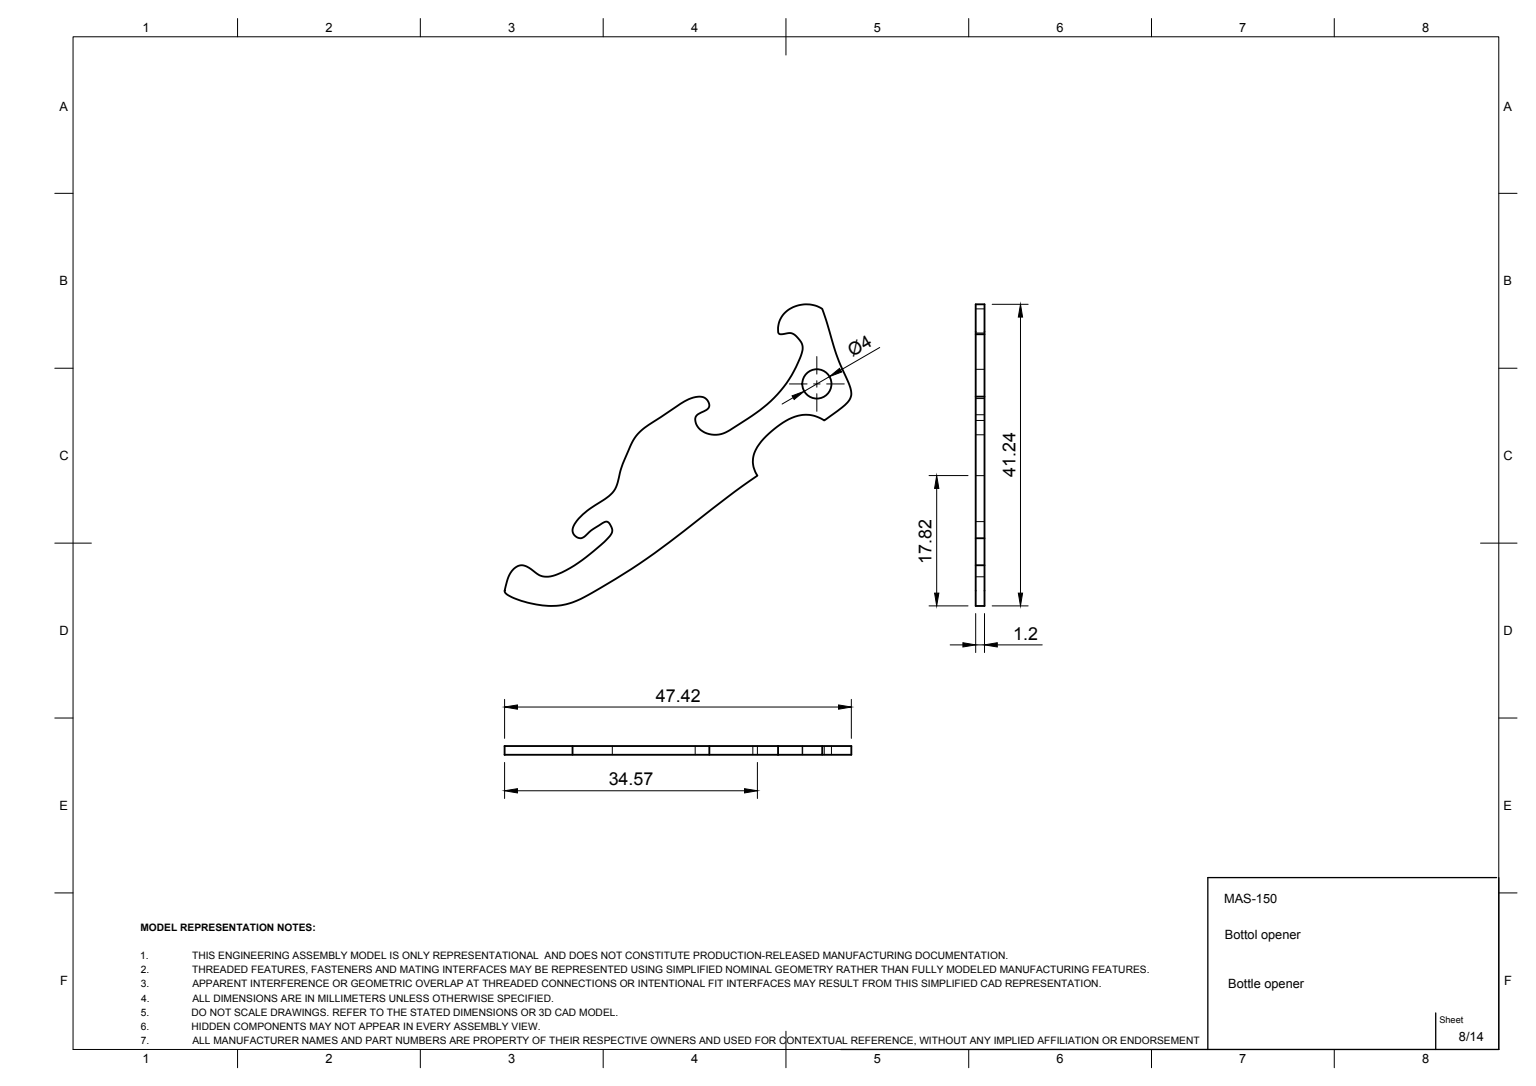
ISO-10303-21;
HEADER;
/* Generated by software containing ST-Developer
 * from STEP Tools, Inc. (www.steptools.com) 
 */

FILE_DESCRIPTION(
/* description */ ('STEP AP203'),
/* implementation_level */ '2;1');

FILE_NAME(
/* name */ 'Bottle opener.step',
/* time_stamp */ '2026-11-08T21:40:52-08:00',
/* author */ (''),
/* organization */ (''),
/* preprocessor_version */ 'ST-DEVELOPER v20.2',
/* originating_system */ 'Autodesk Translation Framework v15.17.0.0',
/* authorisation */ '');

FILE_SCHEMA (('AUTOMOTIVE_DESIGN { 1 0 10303 214 3 1 1 }'));
ENDSEC;

DATA;
#10=MECHANICAL_DESIGN_GEOMETRIC_PRESENTATION_REPRESENTATION('',(#190),#12137);
#128=B_SPLINE_CURVE_WITH_KNOTS('',3,(#11775,#11776,#11777,#11778,#11779,
#11780,#11781,#11782,#11783,#11784,#11785,#11786,#11787,#11788,#11789,#11790,
#11791,#11792,#11793,#11794,#11795,#11796,#11797,#11798,#11799,#11800,#11801,
#11802,#11803,#11804,#11805,#11806,#11807,#11808,#11809,#11810,#11811,#11812,
#11813,#11814,#11815,#11816,#11817,#11818),.UNSPECIFIED.,.F.,.F.,(4,1,1,
1,1,1,1,1,1,1,1,1,1,1,1,1,1,1,1,1,1,1,1,1,1,1,1,1,1,1,1,1,1,1,1,1,1,1,1,
1,1,4),(0.,0.0155086969164078,0.0371731810819821,0.0514015376726156,0.0721494932844473,
0.0879462852339701,0.102136934793609,0.118096046183078,0.19862023937012,
0.220465782155634,0.23365418085247,0.241548051822006,0.250379403180355,
0.265039089454663,0.283941482221575,0.302847655089067,0.314345531734621,
0.357463421988275,0.386547700128901,0.416631362178992,0.447827251721429,
0.480835486339271,0.507932786796811,0.529341861229807,0.553738573125003,
0.594012510221834,0.628912316880978,0.64568724667197,0.66015205447044,0.674349782601168,
0.687580075802142,0.700468884473892,0.724215901035998,0.747660515873313,
0.770169322257755,0.837047273198873,0.898018999477543,0.927421383188233,
0.952466294986228,0.96568815856341,0.980894474823001,1.),.UNSPECIFIED.);
#129=B_SPLINE_CURVE_WITH_KNOTS('',3,(#11822,#11823,#11824,#11825,#11826,
#11827,#11828,#11829,#11830,#11831,#11832,#11833,#11834,#11835,#11836,#11837,
#11838,#11839,#11840,#11841,#11842,#11843,#11844,#11845,#11846,#11847,#11848,
#11849,#11850,#11851,#11852,#11853,#11854,#11855,#11856,#11857,#11858,#11859,
#11860,#11861,#11862,#11863,#11864,#11865),.UNSPECIFIED.,.F.,.F.,(4,1,1,
1,1,1,1,1,1,1,1,1,1,1,1,1,1,1,1,1,1,1,1,1,1,1,1,1,1,1,1,1,1,1,1,1,1,1,1,
1,1,4),(0.,0.0155086969164078,0.0371731810819821,0.0514015376726156,0.0721494932844473,
0.0879462852339701,0.102136934793609,0.118096046183078,0.19862023937012,
0.220465782155634,0.23365418085247,0.241548051822006,0.250379403180355,
0.265039089454663,0.283941482221575,0.302847655089067,0.314345531734621,
0.357463421988275,0.386547700128901,0.416631362178992,0.447827251721429,
0.480835486339271,0.507932786796811,0.529341861229807,0.553738573125003,
0.594012510221834,0.628912316880978,0.64568724667197,0.66015205447044,0.674349782601168,
0.687580075802142,0.700468884473892,0.724215901035998,0.747660515873313,
0.770169322257755,0.837047273198873,0.898018999477543,0.927421383188233,
0.952466294986228,0.96568815856341,0.980894474823001,1.),.UNSPECIFIED.);
#130=B_SPLINE_CURVE_WITH_KNOTS('',3,(#11878,#11879,#11880,#11881),
 .UNSPECIFIED.,.F.,.F.,(4,4),(0.,1.),.UNSPECIFIED.);
#131=B_SPLINE_CURVE_WITH_KNOTS('',3,(#11884,#11885,#11886,#11887),
 .UNSPECIFIED.,.F.,.F.,(4,4),(0.,1.),.UNSPECIFIED.);
#132=B_SPLINE_CURVE_WITH_KNOTS('',3,(#11901,#11902,#11903,#11904,#11905,
#11906),.UNSPECIFIED.,.F.,.F.,(4,1,1,4),(0.,0.470503009353909,0.684670022609357,
1.),.UNSPECIFIED.);
#133=B_SPLINE_CURVE_WITH_KNOTS('',3,(#11909,#11910,#11911,#11912,#11913,
#11914),.UNSPECIFIED.,.F.,.F.,(4,1,1,4),(0.,0.470503009353909,0.684670022609357,
1.),.UNSPECIFIED.);
#134=B_SPLINE_CURVE_WITH_KNOTS('',3,(#11926,#11927,#11928,#11929,#11930),
 .UNSPECIFIED.,.F.,.F.,(4,1,4),(0.,0.519782906107891,1.),.UNSPECIFIED.);
#135=B_SPLINE_CURVE_WITH_KNOTS('',3,(#11933,#11934,#11935,#11936,#11937),
 .UNSPECIFIED.,.F.,.F.,(4,1,4),(0.,0.519782906107891,1.),.UNSPECIFIED.);
#136=B_SPLINE_CURVE_WITH_KNOTS('',3,(#11952,#11953,#11954,#11955,#11956,
#11957,#11958),.UNSPECIFIED.,.F.,.F.,(4,1,1,1,4),(0.,0.490961406160804,
0.688676820334042,0.846051539210629,1.),.UNSPECIFIED.);
#137=B_SPLINE_CURVE_WITH_KNOTS('',3,(#11959,#11960,#11961,#11962,#11963,
#11964,#11965),.UNSPECIFIED.,.F.,.F.,(4,1,1,1,4),(0.,0.490961406160804,
0.688676820334042,0.846051539210629,1.),.UNSPECIFIED.);
#156=B_SPLINE_SURFACE_WITH_KNOTS('',3,1,((#11685,#11686),(#11687,#11688),
(#11689,#11690),(#11691,#11692),(#11693,#11694),(#11695,#11696),(#11697,
#11698),(#11699,#11700),(#11701,#11702),(#11703,#11704),(#11705,#11706),
(#11707,#11708),(#11709,#11710),(#11711,#11712),(#11713,#11714),(#11715,
#11716),(#11717,#11718),(#11719,#11720),(#11721,#11722),(#11723,#11724),
(#11725,#11726),(#11727,#11728),(#11729,#11730),(#11731,#11732),(#11733,
#11734),(#11735,#11736),(#11737,#11738),(#11739,#11740),(#11741,#11742),
(#11743,#11744),(#11745,#11746),(#11747,#11748),(#11749,#11750),(#11751,
#11752),(#11753,#11754),(#11755,#11756),(#11757,#11758),(#11759,#11760),
(#11761,#11762),(#11763,#11764),(#11765,#11766),(#11767,#11768),(#11769,
#11770),(#11771,#11772)),.UNSPECIFIED.,.F.,.F.,.F.,(4,1,1,1,1,1,1,1,1,1,
1,1,1,1,1,1,1,1,1,1,1,1,1,1,1,1,1,1,1,1,1,1,1,1,1,1,1,1,1,1,1,4),(2,2),
(0.,0.0155086969164078,0.0371731810819821,0.0514015376726156,0.0721494932844473,
0.0879462852339701,0.102136934793609,0.118096046183078,0.19862023937012,
0.220465782155634,0.23365418085247,0.241548051822006,0.250379403180355,
0.265039089454663,0.283941482221575,0.302847655089067,0.314345531734621,
0.357463421988275,0.386547700128901,0.416631362178992,0.447827251721429,
0.480835486339271,0.507932786796811,0.529341861229807,0.553738573125003,
0.594012510221834,0.628912316880978,0.64568724667197,0.66015205447044,0.674349782601168,
0.687580075802142,0.700468884473892,0.724215901035998,0.747660515873313,
0.770169322257755,0.837047273198873,0.898018999477543,0.927421383188233,
0.952466294986228,0.96568815856341,0.980894474823001,1.),(0.,0.1728),
 .UNSPECIFIED.);
#157=B_SPLINE_SURFACE_WITH_KNOTS('',3,1,((#11867,#11868),(#11869,#11870),
(#11871,#11872),(#11873,#11874),(#11875,#11876)),.UNSPECIFIED.,.F.,.F.,
 .F.,(4,1,4),(2,2),(0.,0.376046516805316,1.),(0.,0.1728),.UNSPECIFIED.);
#158=B_SPLINE_SURFACE_WITH_KNOTS('',3,1,((#11888,#11889),(#11890,#11891),
(#11892,#11893),(#11894,#11895),(#11896,#11897),(#11898,#11899)),
 .UNSPECIFIED.,.F.,.F.,.F.,(4,1,1,4),(2,2),(0.,0.470503009353909,0.684670022609357,
1.),(0.,0.1728),.UNSPECIFIED.);
#159=B_SPLINE_SURFACE_WITH_KNOTS('',3,1,((#11915,#11916),(#11917,#11918),
(#11919,#11920),(#11921,#11922),(#11923,#11924)),.UNSPECIFIED.,.F.,.F.,
 .F.,(4,1,4),(2,2),(0.,0.519782906107891,1.),(0.,0.1728),.UNSPECIFIED.);
#160=B_SPLINE_SURFACE_WITH_KNOTS('',3,1,((#11938,#11939),(#11940,#11941),
(#11942,#11943),(#11944,#11945),(#11946,#11947),(#11948,#11949),(#11950,
#11951)),.UNSPECIFIED.,.F.,.F.,.F.,(4,1,1,1,4),(2,2),(0.,0.490961406160804,
0.688676820334042,0.846051539210629,1.),(0.,0.1728),.UNSPECIFIED.);
#168=SHAPE_REPRESENTATION_RELATIONSHIP('SRR','None',#12192,#179);
#179=ADVANCED_BREP_SHAPE_REPRESENTATION('',(#201),#12133);
#190=STYLED_ITEM('',(#12253),#201);
#201=MANIFOLD_SOLID_BREP('Body1',#1835);
#221=FACE_BOUND('',#696,.T.);
#222=FACE_BOUND('',#698,.T.);
#263=PLANE('',#2078);
#264=PLANE('',#2079);
#340=LINE('',#11683,#434);
#341=LINE('',#11820,#435);
#342=LINE('',#11866,#436);
#343=LINE('',#11883,#437);
#344=LINE('',#11908,#438);
#345=LINE('',#11932,#439);
#434=VECTOR('',#2456,2.00000000000001);
#435=VECTOR('',#2459,1000.);
#436=VECTOR('',#2460,1000.);
#437=VECTOR('',#2461,1000.);
#438=VECTOR('',#2462,1000.);
#439=VECTOR('',#2463,1000.);
#477=CYLINDRICAL_SURFACE('',#2075,2.00000000000001);
#563=FACE_OUTER_BOUND('',#689,.T.);
#564=FACE_OUTER_BOUND('',#690,.T.);
#565=FACE_OUTER_BOUND('',#691,.T.);
#566=FACE_OUTER_BOUND('',#692,.T.);
#567=FACE_OUTER_BOUND('',#693,.T.);
#568=FACE_OUTER_BOUND('',#694,.T.);
#569=FACE_OUTER_BOUND('',#695,.T.);
#570=FACE_OUTER_BOUND('',#697,.T.);
#689=EDGE_LOOP('',(#1551,#1552,#1553,#1554));
#690=EDGE_LOOP('',(#1555,#1556,#1557,#1558));
#691=EDGE_LOOP('',(#1559,#1560,#1561,#1562));
#692=EDGE_LOOP('',(#1563,#1564,#1565,#1566));
#693=EDGE_LOOP('',(#1567,#1568,#1569,#1570));
#694=EDGE_LOOP('',(#1571,#1572,#1573,#1574));
#695=EDGE_LOOP('',(#1575,#1576,#1577,#1578,#1579));
#696=EDGE_LOOP('',(#1580));
#697=EDGE_LOOP('',(#1581,#1582,#1583,#1584,#1585));
#698=EDGE_LOOP('',(#1586));
#786=CIRCLE('',#2076,2.00000000000001);
#787=CIRCLE('',#2077,2.00000000000001);
#931=VERTEX_POINT('',#11680);
#932=VERTEX_POINT('',#11682);
#933=VERTEX_POINT('',#11773);
#934=VERTEX_POINT('',#11774);
#935=VERTEX_POINT('',#11819);
#936=VERTEX_POINT('',#11821);
#937=VERTEX_POINT('',#11877);
#938=VERTEX_POINT('',#11882);
#939=VERTEX_POINT('',#11900);
#940=VERTEX_POINT('',#11907);
#941=VERTEX_POINT('',#11925);
#942=VERTEX_POINT('',#11931);
#1145=EDGE_CURVE('',#931,#931,#786,.T.);
#1146=EDGE_CURVE('',#931,#932,#340,.T.);
#1147=EDGE_CURVE('',#932,#932,#787,.T.);
#1148=EDGE_CURVE('',#933,#934,#128,.T.);
#1149=EDGE_CURVE('',#935,#934,#341,.T.);
#1150=EDGE_CURVE('',#936,#935,#129,.T.);
#1151=EDGE_CURVE('',#936,#933,#342,.T.);
#1152=EDGE_CURVE('',#934,#937,#130,.T.);
#1153=EDGE_CURVE('',#938,#937,#343,.T.);
#1154=EDGE_CURVE('',#935,#938,#131,.T.);
#1155=EDGE_CURVE('',#937,#939,#132,.T.);
#1156=EDGE_CURVE('',#940,#939,#344,.T.);
#1157=EDGE_CURVE('',#938,#940,#133,.T.);
#1158=EDGE_CURVE('',#939,#941,#134,.T.);
#1159=EDGE_CURVE('',#942,#941,#345,.T.);
#1160=EDGE_CURVE('',#940,#942,#135,.T.);
#1161=EDGE_CURVE('',#941,#933,#136,.T.);
#1162=EDGE_CURVE('',#942,#936,#137,.T.);
#1551=ORIENTED_EDGE('',*,*,#1145,.F.);
#1552=ORIENTED_EDGE('',*,*,#1146,.T.);
#1553=ORIENTED_EDGE('',*,*,#1147,.T.);
#1554=ORIENTED_EDGE('',*,*,#1146,.F.);
#1555=ORIENTED_EDGE('',*,*,#1148,.T.);
#1556=ORIENTED_EDGE('',*,*,#1149,.F.);
#1557=ORIENTED_EDGE('',*,*,#1150,.F.);
#1558=ORIENTED_EDGE('',*,*,#1151,.T.);
#1559=ORIENTED_EDGE('',*,*,#1152,.T.);
#1560=ORIENTED_EDGE('',*,*,#1153,.F.);
#1561=ORIENTED_EDGE('',*,*,#1154,.F.);
#1562=ORIENTED_EDGE('',*,*,#1149,.T.);
#1563=ORIENTED_EDGE('',*,*,#1155,.T.);
#1564=ORIENTED_EDGE('',*,*,#1156,.F.);
#1565=ORIENTED_EDGE('',*,*,#1157,.F.);
#1566=ORIENTED_EDGE('',*,*,#1153,.T.);
#1567=ORIENTED_EDGE('',*,*,#1158,.T.);
#1568=ORIENTED_EDGE('',*,*,#1159,.F.);
#1569=ORIENTED_EDGE('',*,*,#1160,.F.);
#1570=ORIENTED_EDGE('',*,*,#1156,.T.);
#1571=ORIENTED_EDGE('',*,*,#1161,.T.);
#1572=ORIENTED_EDGE('',*,*,#1151,.F.);
#1573=ORIENTED_EDGE('',*,*,#1162,.F.);
#1574=ORIENTED_EDGE('',*,*,#1159,.T.);
#1575=ORIENTED_EDGE('',*,*,#1150,.T.);
#1576=ORIENTED_EDGE('',*,*,#1154,.T.);
#1577=ORIENTED_EDGE('',*,*,#1157,.T.);
#1578=ORIENTED_EDGE('',*,*,#1160,.T.);
#1579=ORIENTED_EDGE('',*,*,#1162,.T.);
#1580=ORIENTED_EDGE('',*,*,#1147,.F.);
#1581=ORIENTED_EDGE('',*,*,#1148,.F.);
#1582=ORIENTED_EDGE('',*,*,#1161,.F.);
#1583=ORIENTED_EDGE('',*,*,#1158,.F.);
#1584=ORIENTED_EDGE('',*,*,#1155,.F.);
#1585=ORIENTED_EDGE('',*,*,#1152,.F.);
#1586=ORIENTED_EDGE('',*,*,#1145,.T.);
#1791=ADVANCED_FACE('',(#563),#477,.F.);
#1792=ADVANCED_FACE('',(#564),#156,.F.);
#1793=ADVANCED_FACE('',(#565),#157,.F.);
#1794=ADVANCED_FACE('',(#566),#158,.F.);
#1795=ADVANCED_FACE('',(#567),#159,.F.);
#1796=ADVANCED_FACE('',(#568),#160,.F.);
#1797=ADVANCED_FACE('',(#569,#221),#263,.T.);
#1798=ADVANCED_FACE('',(#570,#222),#264,.F.);
#1835=CLOSED_SHELL('',(#1791,#1792,#1793,#1794,#1795,#1796,#1797,#1798));
#2074=AXIS2_PLACEMENT_3D('',#11678,#2450,#2451);
#2075=AXIS2_PLACEMENT_3D('',#11679,#2452,#2453);
#2076=AXIS2_PLACEMENT_3D('',#11681,#2454,#2455);
#2077=AXIS2_PLACEMENT_3D('',#11684,#2457,#2458);
#2078=AXIS2_PLACEMENT_3D('',#11966,#2464,#2465);
#2079=AXIS2_PLACEMENT_3D('',#11967,#2466,#2467);
#2450=DIRECTION('axis',(0.,0.,1.));
#2451=DIRECTION('refdir',(1.,0.,0.));
#2452=DIRECTION('center_axis',(-1.77763333866942E-31,1.,8.62816615085482E-32));
#2453=DIRECTION('ref_axis',(2.87582171275097E-62,-8.62816615085482E-32,
1.));
#2454=DIRECTION('center_axis',(-1.77763333866942E-31,1.,8.62816615085482E-32));
#2455=DIRECTION('ref_axis',(2.87582171275097E-62,-8.62816615085482E-32,
1.));
#2456=DIRECTION('',(-1.77763333866942E-31,1.,8.62816615085482E-32));
#2457=DIRECTION('center_axis',(-1.77763333866942E-31,1.,8.62816615085482E-32));
#2458=DIRECTION('ref_axis',(1.53377158013385E-62,-8.62816615085482E-32,
1.));
#2459=DIRECTION('',(1.77763333866942E-31,-1.,-8.62816615085482E-32));
#2460=DIRECTION('',(1.77763333866942E-31,-1.,-8.62816615085482E-32));
#2461=DIRECTION('',(1.77763333866942E-31,-1.,-8.62816615085482E-32));
#2462=DIRECTION('',(1.77763333866942E-31,-1.,-8.62816615085482E-32));
#2463=DIRECTION('',(1.77763333866942E-31,-1.,-8.62816615085482E-32));
#2464=DIRECTION('center_axis',(-1.77763333866942E-31,1.,-7.54964538199795E-32));
#2465=DIRECTION('ref_axis',(2.67771827758074E-79,7.54964538199795E-32,1.));
#2466=DIRECTION('center_axis',(-1.77763333866942E-31,1.,-7.54964538199795E-32));
#2467=DIRECTION('ref_axis',(2.67771827758074E-79,7.54964538199795E-32,1.));
#11678=CARTESIAN_POINT('',(0.,0.,0.));
#11679=CARTESIAN_POINT('Origin',(22.9603057217174,0.,-2.33853588412019));
#11680=CARTESIAN_POINT('',(22.9603057217174,1.72563323017097E-31,-4.3385358841202));
#11681=CARTESIAN_POINT('Origin',(22.9603057217174,0.,-2.33853588412019));
#11682=CARTESIAN_POINT('',(22.9603057217174,1.2,-4.3385358841202));
#11683=CARTESIAN_POINT('',(22.9603057217174,1.72563323017097E-31,-4.3385358841202));
#11684=CARTESIAN_POINT('Origin',(22.9603057217174,1.2,-2.33853588412019));
#11685=CARTESIAN_POINT('Ctrl Pts',(-28.2500418808544,1.2,-2.07888836971772));
#11686=CARTESIAN_POINT('Ctrl Pts',(-28.2500418808544,-0.527999999999998,
-2.07888836971772));
#11687=CARTESIAN_POINT('Ctrl Pts',(-27.9613439331009,1.2,-1.81555449964671));
#11688=CARTESIAN_POINT('Ctrl Pts',(-27.9613439331009,-0.527999999999998,
-1.81555449964671));
#11689=CARTESIAN_POINT('Ctrl Pts',(-27.180603234679,1.2,-1.04385836116026));
#11690=CARTESIAN_POINT('Ctrl Pts',(-27.180603234679,-0.527999999999998,
-1.04385836116026));
#11691=CARTESIAN_POINT('Ctrl Pts',(-25.9983030006616,1.2,-0.24124876693352));
#11692=CARTESIAN_POINT('Ctrl Pts',(-25.9983030006616,-0.527999999999998,
-0.24124876693352));
#11693=CARTESIAN_POINT('Ctrl Pts',(-24.2346861695509,1.2,-0.210983790359477));
#11694=CARTESIAN_POINT('Ctrl Pts',(-24.2346861695509,-0.527999999999998,
-0.210983790359477));
#11695=CARTESIAN_POINT('Ctrl Pts',(-23.517870169039,1.2,-1.68305705631707));
#11696=CARTESIAN_POINT('Ctrl Pts',(-23.517870169039,-0.527999999999998,
-1.68305705631707));
#11697=CARTESIAN_POINT('Ctrl Pts',(-23.2233109717715,1.2,-3.05602157557454));
#11698=CARTESIAN_POINT('Ctrl Pts',(-23.2233109717715,-0.527999999999998,
-3.05602157557454));
#11699=CARTESIAN_POINT('Ctrl Pts',(-22.1784263046757,1.2,-3.93337248074442));
#11700=CARTESIAN_POINT('Ctrl Pts',(-22.1784263046757,-0.527999999999998,
-3.93337248074442));
#11701=CARTESIAN_POINT('Ctrl Pts',(-19.19441431546,1.2,-4.74815122044273));
#11702=CARTESIAN_POINT('Ctrl Pts',(-19.19441431546,-0.527999999999998,-4.74815122044273));
#11703=CARTESIAN_POINT('Ctrl Pts',(-15.7509580358841,1.2,-4.44216895895114));
#11704=CARTESIAN_POINT('Ctrl Pts',(-15.7509580358841,-0.527999999999998,
-4.44216895895114));
#11705=CARTESIAN_POINT('Ctrl Pts',(-12.7021174144063,1.2,-4.06331666259747));
#11706=CARTESIAN_POINT('Ctrl Pts',(-12.7021174144063,-0.527999999999998,
-4.06331666259747));
#11707=CARTESIAN_POINT('Ctrl Pts',(-11.3962777017639,1.2,-3.64648316501468));
#11708=CARTESIAN_POINT('Ctrl Pts',(-11.3962777017639,-0.527999999999998,
-3.64648316501468));
#11709=CARTESIAN_POINT('Ctrl Pts',(-11.2344759364774,1.2,-2.80455171594097));
#11710=CARTESIAN_POINT('Ctrl Pts',(-11.2344759364774,-0.527999999999998,
-2.80455171594097));
#11711=CARTESIAN_POINT('Ctrl Pts',(-11.1732737269437,1.2,-1.7662619507528));
#11712=CARTESIAN_POINT('Ctrl Pts',(-11.1732737269437,-0.527999999999998,
-1.7662619507528));
#11713=CARTESIAN_POINT('Ctrl Pts',(-12.7612302838612,1.2,-1.89361059761595));
#11714=CARTESIAN_POINT('Ctrl Pts',(-12.7612302838612,-0.527999999999998,
-1.89361059761595));
#11715=CARTESIAN_POINT('Ctrl Pts',(-13.9972305202523,1.2,-1.67844839769156));
#11716=CARTESIAN_POINT('Ctrl Pts',(-13.9972305202523,-0.527999999999998,
-1.67844839769156));
#11717=CARTESIAN_POINT('Ctrl Pts',(-15.6400181726054,1.2,-2.29491586659866));
#11718=CARTESIAN_POINT('Ctrl Pts',(-15.6400181726054,-0.527999999999998,
-2.29491586659866));
#11719=CARTESIAN_POINT('Ctrl Pts',(-16.7051564115516,1.2,0.0418535888021335));
#11720=CARTESIAN_POINT('Ctrl Pts',(-16.7051564115516,-0.527999999999998,
0.0418535888021335));
#11721=CARTESIAN_POINT('Ctrl Pts',(-13.0664970088623,1.2,0.88071809162054));
#11722=CARTESIAN_POINT('Ctrl Pts',(-13.0664970088623,-0.527999999999998,
0.88071809162054));
#11723=CARTESIAN_POINT('Ctrl Pts',(-10.5984973129989,1.2,0.680667707785562));
#11724=CARTESIAN_POINT('Ctrl Pts',(-10.5984973129989,-0.527999999999998,
0.680667707785562));
#11725=CARTESIAN_POINT('Ctrl Pts',(-7.82942308877726,1.2,0.695565326486597));
#11726=CARTESIAN_POINT('Ctrl Pts',(-7.82942308877726,-0.527999999999998,
0.695565326486597));
#11727=CARTESIAN_POINT('Ctrl Pts',(-6.07620266579566,1.2,2.85997113365485));
#11728=CARTESIAN_POINT('Ctrl Pts',(-6.07620266579566,-0.527999999999998,
2.85997113365485));
#11729=CARTESIAN_POINT('Ctrl Pts',(-3.9066933893458,1.2,4.14091208560258));
#11730=CARTESIAN_POINT('Ctrl Pts',(-3.9066933893458,-0.527999999999998,
4.14091208560258));
#11731=CARTESIAN_POINT('Ctrl Pts',(-2.0279101215411,1.2,5.46819912841997));
#11732=CARTESIAN_POINT('Ctrl Pts',(-2.0279101215411,-0.527999999999998,
5.46819912841997));
#11733=CARTESIAN_POINT('Ctrl Pts',(0.00386116068497311,1.2,5.86471136207473));
#11734=CARTESIAN_POINT('Ctrl Pts',(0.00386116068497311,-0.527999999999998,
5.86471136207473));
#11735=CARTESIAN_POINT('Ctrl Pts',(2.39576994688095,1.2,5.73794061249253));
#11736=CARTESIAN_POINT('Ctrl Pts',(2.39576994688095,-0.527999999999998,
5.73794061249253));
#11737=CARTESIAN_POINT('Ctrl Pts',(5.15590481840992,1.2,5.78580883625202));
#11738=CARTESIAN_POINT('Ctrl Pts',(5.15590481840992,-0.527999999999998,
5.78580883625202));
#11739=CARTESIAN_POINT('Ctrl Pts',(7.73518803149787,1.2,5.79127386586831));
#11740=CARTESIAN_POINT('Ctrl Pts',(7.73518803149787,-0.527999999999998,
5.79127386586831));
#11741=CARTESIAN_POINT('Ctrl Pts',(9.45734572072178,1.2,4.67363967594622));
#11742=CARTESIAN_POINT('Ctrl Pts',(9.45734572072178,-0.527999999999998,
4.67363967594622));
#11743=CARTESIAN_POINT('Ctrl Pts',(9.17706365495184,1.2,2.96306509995752));
#11744=CARTESIAN_POINT('Ctrl Pts',(9.17706365495184,-0.527999999999998,
2.96306509995752));
#11745=CARTESIAN_POINT('Ctrl Pts',(7.81796360098053,1.2,3.18513163158631));
#11746=CARTESIAN_POINT('Ctrl Pts',(7.81796360098053,-0.527999999999998,
3.18513163158631));
#11747=CARTESIAN_POINT('Ctrl Pts',(6.59699346312693,1.2,3.38520430984983));
#11748=CARTESIAN_POINT('Ctrl Pts',(6.59699346312693,-0.527999999999998,
3.38520430984983));
#11749=CARTESIAN_POINT('Ctrl Pts',(5.93021602745299,1.2,1.85802575211607));
#11750=CARTESIAN_POINT('Ctrl Pts',(5.93021602745299,-0.527999999999998,
1.85802575211607));
#11751=CARTESIAN_POINT('Ctrl Pts',(6.62071623580517,1.2,0.188782666588939));
#11752=CARTESIAN_POINT('Ctrl Pts',(6.62071623580517,-0.527999999999998,
0.188782666588939));
#11753=CARTESIAN_POINT('Ctrl Pts',(8.32325294445203,1.2,-0.970953886492654));
#11754=CARTESIAN_POINT('Ctrl Pts',(8.32325294445203,-0.527999999999998,
-0.970953886492654));
#11755=CARTESIAN_POINT('Ctrl Pts',(11.5219206080117,1.2,-0.983963678117389));
#11756=CARTESIAN_POINT('Ctrl Pts',(11.5219206080117,-0.527999999999998,
-0.983963678117389));
#11757=CARTESIAN_POINT('Ctrl Pts',(15.6615569014707,1.2,-1.18440486857005));
#11758=CARTESIAN_POINT('Ctrl Pts',(15.6615569014707,-0.527999999999998,
-1.18440486857005));
#11759=CARTESIAN_POINT('Ctrl Pts',(20.0374444881341,1.2,0.065252622484184));
#11760=CARTESIAN_POINT('Ctrl Pts',(20.0374444881341,-0.527999999999998,
0.065252622484184));
#11761=CARTESIAN_POINT('Ctrl Pts',(22.6903241895972,1.2,1.63809077991409));
#11762=CARTESIAN_POINT('Ctrl Pts',(22.6903241895972,-0.527999999999998,
1.63809077991409));
#11763=CARTESIAN_POINT('Ctrl Pts',(24.4689719714588,1.2,2.87083584760694));
#11764=CARTESIAN_POINT('Ctrl Pts',(24.4689719714588,-0.527999999999998,
2.87083584760694));
#11765=CARTESIAN_POINT('Ctrl Pts',(24.3083816239237,1.2,4.43315301466272));
#11766=CARTESIAN_POINT('Ctrl Pts',(24.3083816239237,-0.527999999999998,
4.43315301466272));
#11767=CARTESIAN_POINT('Ctrl Pts',(24.0522028467612,1.2,5.77390669222975));
#11768=CARTESIAN_POINT('Ctrl Pts',(24.0522028467612,-0.527999999999998,
5.77390669222975));
#11769=CARTESIAN_POINT('Ctrl Pts',(22.2137376328105,1.2,5.96195834426836));
#11770=CARTESIAN_POINT('Ctrl Pts',(22.2137376328105,-0.527999999999998,
5.96195834426836));
#11771=CARTESIAN_POINT('Ctrl Pts',(22.5278884970739,1.2,6.53446701068235));
#11772=CARTESIAN_POINT('Ctrl Pts',(22.5278884970739,-0.527999999999998,
6.53446701068235));
#11773=CARTESIAN_POINT('',(-28.2500418808543,0.,-2.07888836971769));
#11774=CARTESIAN_POINT('',(22.5278884970739,0.,6.53446701068235));
#11775=CARTESIAN_POINT('Ctrl Pts',(-28.2500418808543,0.,-2.07888836971769));
#11776=CARTESIAN_POINT('Ctrl Pts',(-27.9613439331009,0.,-1.81555449964671));
#11777=CARTESIAN_POINT('Ctrl Pts',(-27.180603234679,0.,-1.04385836116026));
#11778=CARTESIAN_POINT('Ctrl Pts',(-25.9983030006616,0.,-0.24124876693352));
#11779=CARTESIAN_POINT('Ctrl Pts',(-24.2346861695509,0.,-0.210983790359477));
#11780=CARTESIAN_POINT('Ctrl Pts',(-23.517870169039,0.,-1.68305705631707));
#11781=CARTESIAN_POINT('Ctrl Pts',(-23.2233109717715,0.,-3.05602157557454));
#11782=CARTESIAN_POINT('Ctrl Pts',(-22.1784263046757,0.,-3.93337248074442));
#11783=CARTESIAN_POINT('Ctrl Pts',(-19.19441431546,0.,-4.74815122044273));
#11784=CARTESIAN_POINT('Ctrl Pts',(-15.7509580358841,0.,-4.44216895895114));
#11785=CARTESIAN_POINT('Ctrl Pts',(-12.7021174144063,0.,-4.06331666259747));
#11786=CARTESIAN_POINT('Ctrl Pts',(-11.3962777017639,0.,-3.64648316501468));
#11787=CARTESIAN_POINT('Ctrl Pts',(-11.2344759364774,0.,-2.80455171594097));
#11788=CARTESIAN_POINT('Ctrl Pts',(-11.1732737269437,0.,-1.7662619507528));
#11789=CARTESIAN_POINT('Ctrl Pts',(-12.7612302838612,0.,-1.89361059761595));
#11790=CARTESIAN_POINT('Ctrl Pts',(-13.9972305202523,0.,-1.67844839769156));
#11791=CARTESIAN_POINT('Ctrl Pts',(-15.6400181726054,0.,-2.29491586659866));
#11792=CARTESIAN_POINT('Ctrl Pts',(-16.7051564115516,0.,0.0418535888021335));
#11793=CARTESIAN_POINT('Ctrl Pts',(-13.0664970088623,0.,0.88071809162054));
#11794=CARTESIAN_POINT('Ctrl Pts',(-10.5984973129989,0.,0.680667707785562));
#11795=CARTESIAN_POINT('Ctrl Pts',(-7.82942308877726,0.,0.695565326486597));
#11796=CARTESIAN_POINT('Ctrl Pts',(-6.07620266579566,0.,2.85997113365485));
#11797=CARTESIAN_POINT('Ctrl Pts',(-3.9066933893458,0.,4.14091208560258));
#11798=CARTESIAN_POINT('Ctrl Pts',(-2.0279101215411,0.,5.46819912841997));
#11799=CARTESIAN_POINT('Ctrl Pts',(0.00386116068497311,0.,5.86471136207473));
#11800=CARTESIAN_POINT('Ctrl Pts',(2.39576994688095,0.,5.73794061249253));
#11801=CARTESIAN_POINT('Ctrl Pts',(5.15590481840992,0.,5.78580883625202));
#11802=CARTESIAN_POINT('Ctrl Pts',(7.73518803149787,0.,5.79127386586831));
#11803=CARTESIAN_POINT('Ctrl Pts',(9.45734572072178,0.,4.67363967594622));
#11804=CARTESIAN_POINT('Ctrl Pts',(9.17706365495184,0.,2.96306509995752));
#11805=CARTESIAN_POINT('Ctrl Pts',(7.81796360098053,0.,3.18513163158631));
#11806=CARTESIAN_POINT('Ctrl Pts',(6.59699346312693,0.,3.38520430984983));
#11807=CARTESIAN_POINT('Ctrl Pts',(5.93021602745299,0.,1.85802575211607));
#11808=CARTESIAN_POINT('Ctrl Pts',(6.62071623580517,0.,0.188782666588939));
#11809=CARTESIAN_POINT('Ctrl Pts',(8.32325294445203,0.,-0.970953886492654));
#11810=CARTESIAN_POINT('Ctrl Pts',(11.5219206080117,0.,-0.983963678117389));
#11811=CARTESIAN_POINT('Ctrl Pts',(15.6615569014707,0.,-1.18440486857005));
#11812=CARTESIAN_POINT('Ctrl Pts',(20.0374444881341,0.,0.065252622484184));
#11813=CARTESIAN_POINT('Ctrl Pts',(22.6903241895972,0.,1.63809077991409));
#11814=CARTESIAN_POINT('Ctrl Pts',(24.4689719714588,0.,2.87083584760694));
#11815=CARTESIAN_POINT('Ctrl Pts',(24.3083816239237,0.,4.43315301466272));
#11816=CARTESIAN_POINT('Ctrl Pts',(24.0522028467612,0.,5.77390669222975));
#11817=CARTESIAN_POINT('Ctrl Pts',(22.2137376328105,0.,5.96195834426836));
#11818=CARTESIAN_POINT('Ctrl Pts',(22.5278884970739,0.,6.53446701068235));
#11819=CARTESIAN_POINT('',(22.5278884970739,1.2,6.53446701068235));
#11820=CARTESIAN_POINT('',(22.5278884970739,1.2,6.53446701068235));
#11821=CARTESIAN_POINT('',(-28.2500418808543,1.2,-2.07888836971769));
#11822=CARTESIAN_POINT('Ctrl Pts',(-28.2500418808543,1.2,-2.07888836971769));
#11823=CARTESIAN_POINT('Ctrl Pts',(-27.9613439331009,1.2,-1.81555449964671));
#11824=CARTESIAN_POINT('Ctrl Pts',(-27.180603234679,1.2,-1.04385836116026));
#11825=CARTESIAN_POINT('Ctrl Pts',(-25.9983030006616,1.2,-0.24124876693352));
#11826=CARTESIAN_POINT('Ctrl Pts',(-24.2346861695509,1.2,-0.210983790359477));
#11827=CARTESIAN_POINT('Ctrl Pts',(-23.517870169039,1.2,-1.68305705631707));
#11828=CARTESIAN_POINT('Ctrl Pts',(-23.2233109717715,1.2,-3.05602157557454));
#11829=CARTESIAN_POINT('Ctrl Pts',(-22.1784263046757,1.2,-3.93337248074442));
#11830=CARTESIAN_POINT('Ctrl Pts',(-19.19441431546,1.2,-4.74815122044273));
#11831=CARTESIAN_POINT('Ctrl Pts',(-15.7509580358841,1.2,-4.44216895895114));
#11832=CARTESIAN_POINT('Ctrl Pts',(-12.7021174144063,1.2,-4.06331666259747));
#11833=CARTESIAN_POINT('Ctrl Pts',(-11.3962777017639,1.2,-3.64648316501468));
#11834=CARTESIAN_POINT('Ctrl Pts',(-11.2344759364774,1.2,-2.80455171594097));
#11835=CARTESIAN_POINT('Ctrl Pts',(-11.1732737269437,1.2,-1.7662619507528));
#11836=CARTESIAN_POINT('Ctrl Pts',(-12.7612302838612,1.2,-1.89361059761595));
#11837=CARTESIAN_POINT('Ctrl Pts',(-13.9972305202523,1.2,-1.67844839769156));
#11838=CARTESIAN_POINT('Ctrl Pts',(-15.6400181726054,1.2,-2.29491586659866));
#11839=CARTESIAN_POINT('Ctrl Pts',(-16.7051564115516,1.2,0.0418535888021335));
#11840=CARTESIAN_POINT('Ctrl Pts',(-13.0664970088623,1.2,0.88071809162054));
#11841=CARTESIAN_POINT('Ctrl Pts',(-10.5984973129989,1.2,0.680667707785562));
#11842=CARTESIAN_POINT('Ctrl Pts',(-7.82942308877726,1.2,0.695565326486597));
#11843=CARTESIAN_POINT('Ctrl Pts',(-6.07620266579566,1.2,2.85997113365485));
#11844=CARTESIAN_POINT('Ctrl Pts',(-3.9066933893458,1.2,4.14091208560258));
#11845=CARTESIAN_POINT('Ctrl Pts',(-2.0279101215411,1.2,5.46819912841997));
#11846=CARTESIAN_POINT('Ctrl Pts',(0.00386116068497311,1.2,5.86471136207473));
#11847=CARTESIAN_POINT('Ctrl Pts',(2.39576994688095,1.2,5.73794061249253));
#11848=CARTESIAN_POINT('Ctrl Pts',(5.15590481840992,1.2,5.78580883625202));
#11849=CARTESIAN_POINT('Ctrl Pts',(7.73518803149787,1.2,5.79127386586831));
#11850=CARTESIAN_POINT('Ctrl Pts',(9.45734572072178,1.2,4.67363967594622));
#11851=CARTESIAN_POINT('Ctrl Pts',(9.17706365495184,1.2,2.96306509995752));
#11852=CARTESIAN_POINT('Ctrl Pts',(7.81796360098053,1.2,3.18513163158631));
#11853=CARTESIAN_POINT('Ctrl Pts',(6.59699346312693,1.2,3.38520430984983));
#11854=CARTESIAN_POINT('Ctrl Pts',(5.93021602745299,1.2,1.85802575211607));
#11855=CARTESIAN_POINT('Ctrl Pts',(6.62071623580517,1.2,0.188782666588939));
#11856=CARTESIAN_POINT('Ctrl Pts',(8.32325294445203,1.2,-0.970953886492654));
#11857=CARTESIAN_POINT('Ctrl Pts',(11.5219206080117,1.2,-0.983963678117389));
#11858=CARTESIAN_POINT('Ctrl Pts',(15.6615569014707,1.2,-1.18440486857005));
#11859=CARTESIAN_POINT('Ctrl Pts',(20.0374444881341,1.2,0.065252622484184));
#11860=CARTESIAN_POINT('Ctrl Pts',(22.6903241895972,1.2,1.63809077991409));
#11861=CARTESIAN_POINT('Ctrl Pts',(24.4689719714588,1.2,2.87083584760694));
#11862=CARTESIAN_POINT('Ctrl Pts',(24.3083816239237,1.2,4.43315301466272));
#11863=CARTESIAN_POINT('Ctrl Pts',(24.0522028467612,1.2,5.77390669222975));
#11864=CARTESIAN_POINT('Ctrl Pts',(22.2137376328105,1.2,5.96195834426836));
#11865=CARTESIAN_POINT('Ctrl Pts',(22.5278884970739,1.2,6.53446701068235));
#11866=CARTESIAN_POINT('',(-28.2500418808543,1.2,-2.07888836971769));
#11867=CARTESIAN_POINT('Ctrl Pts',(22.5278884970739,1.2,6.53446701068235));
#11868=CARTESIAN_POINT('Ctrl Pts',(22.5278884970739,-0.528,6.53446701068235));
#11869=CARTESIAN_POINT('Ctrl Pts',(23.1169295329987,1.2,7.60793564089319));
#11870=CARTESIAN_POINT('Ctrl Pts',(23.1169295329987,-0.528,7.60793564089319));
#11871=CARTESIAN_POINT('Ctrl Pts',(25.6536230216728,1.2,8.99671226634374));
#11872=CARTESIAN_POINT('Ctrl Pts',(25.6536230216728,-0.528,8.99671226634374));
#11873=CARTESIAN_POINT('Ctrl Pts',(28.6313409150419,1.2,7.38059742138985));
#11874=CARTESIAN_POINT('Ctrl Pts',(28.6313409150419,-0.528,7.38059742138985));
#11875=CARTESIAN_POINT('Ctrl Pts',(29.2791218831689,1.2,5.77930198399101));
#11876=CARTESIAN_POINT('Ctrl Pts',(29.2791218831689,-0.528,5.77930198399101));
#11877=CARTESIAN_POINT('',(29.2791218831689,0.,5.77930198399101));
#11878=CARTESIAN_POINT('Ctrl Pts',(22.5278884970739,0.,6.53446701068235));
#11879=CARTESIAN_POINT('Ctrl Pts',(24.0942932092593,0.,9.38908361325172));
#11880=CARTESIAN_POINT('Ctrl Pts',(28.2409339643995,0.,8.34567188259311));
#11881=CARTESIAN_POINT('Ctrl Pts',(29.2791218831689,0.,5.77930198399101));
#11882=CARTESIAN_POINT('',(29.2791218831689,1.2,5.77930198399101));
#11883=CARTESIAN_POINT('',(29.2791218831689,1.2,5.77930198399101));
#11884=CARTESIAN_POINT('Ctrl Pts',(22.5278884970739,1.2,6.53446701068235));
#11885=CARTESIAN_POINT('Ctrl Pts',(24.0942932092593,1.2,9.38908361325172));
#11886=CARTESIAN_POINT('Ctrl Pts',(28.2409339643995,1.2,8.34567188259311));
#11887=CARTESIAN_POINT('Ctrl Pts',(29.2791218831689,1.2,5.77930198399101));
#11888=CARTESIAN_POINT('Ctrl Pts',(29.2791218831689,1.2,5.77930198399101));
#11889=CARTESIAN_POINT('Ctrl Pts',(29.2791218831689,-0.528,5.77930198399101));
#11890=CARTESIAN_POINT('Ctrl Pts',(28.6578105275465,1.2,2.99017303105976));
#11891=CARTESIAN_POINT('Ctrl Pts',(28.6578105275465,-0.528,2.99017303105976));
#11892=CARTESIAN_POINT('Ctrl Pts',(27.094379352357,1.2,-0.177553803652863));
#11893=CARTESIAN_POINT('Ctrl Pts',(27.094379352357,-0.528,-0.177553803652863));
#11894=CARTESIAN_POINT('Ctrl Pts',(26.5382228845289,1.2,-7.0166851266602));
#11895=CARTESIAN_POINT('Ctrl Pts',(26.5382228845289,-0.528,-7.0166851266602));
#11896=CARTESIAN_POINT('Ctrl Pts',(24.629125296679,1.2,-6.94685713119016));
#11897=CARTESIAN_POINT('Ctrl Pts',(24.629125296679,-0.528,-6.94685713119016));
#11898=CARTESIAN_POINT('Ctrl Pts',(21.0225256793385,1.2,-7.04790997553116));
#11899=CARTESIAN_POINT('Ctrl Pts',(21.0225256793385,-0.528,-7.04790997553116));
#11900=CARTESIAN_POINT('',(21.0225256793385,0.,-7.04790997553116));
#11901=CARTESIAN_POINT('Ctrl Pts',(29.2791218831689,0.,5.77930198399101));
#11902=CARTESIAN_POINT('Ctrl Pts',(28.6578105275465,0.,2.99017303105976));
#11903=CARTESIAN_POINT('Ctrl Pts',(27.094379352357,0.,-0.177553803652863));
#11904=CARTESIAN_POINT('Ctrl Pts',(26.5382228845289,0.,-7.0166851266602));
#11905=CARTESIAN_POINT('Ctrl Pts',(24.629125296679,0.,-6.94685713119016));
#11906=CARTESIAN_POINT('Ctrl Pts',(21.0225256793385,0.,-7.04790997553116));
#11907=CARTESIAN_POINT('',(21.0225256793385,1.2,-7.04790997553116));
#11908=CARTESIAN_POINT('',(21.0225256793385,1.2,-7.04790997553116));
#11909=CARTESIAN_POINT('Ctrl Pts',(29.2791218831689,1.2,5.77930198399101));
#11910=CARTESIAN_POINT('Ctrl Pts',(28.6578105275465,1.2,2.99017303105976));
#11911=CARTESIAN_POINT('Ctrl Pts',(27.094379352357,1.2,-0.177553803652863));
#11912=CARTESIAN_POINT('Ctrl Pts',(26.5382228845289,1.2,-7.0166851266602));
#11913=CARTESIAN_POINT('Ctrl Pts',(24.629125296679,1.2,-6.94685713119016));
#11914=CARTESIAN_POINT('Ctrl Pts',(21.0225256793385,1.2,-7.04790997553116));
#11915=CARTESIAN_POINT('Ctrl Pts',(21.0225256793385,1.2,-7.04790997553116));
#11916=CARTESIAN_POINT('Ctrl Pts',(21.0225256793385,-0.528,-7.04790997553116));
#11917=CARTESIAN_POINT('Ctrl Pts',(19.8072013377325,1.2,-4.22629716477465));
#11918=CARTESIAN_POINT('Ctrl Pts',(19.8072013377325,-0.528,-4.22629716477465));
#11919=CARTESIAN_POINT('Ctrl Pts',(14.6387365156322,1.2,-3.68706222835893));
#11920=CARTESIAN_POINT('Ctrl Pts',(14.6387365156322,-0.528,-3.68706222835893));
#11921=CARTESIAN_POINT('Ctrl Pts',(9.29823038687031,1.2,-5.29769106666559));
#11922=CARTESIAN_POINT('Ctrl Pts',(9.29823038687031,-0.528,-5.29769106666559));
#11923=CARTESIAN_POINT('Ctrl Pts',(9.22738824529516,1.2,-8.22742371893551));
#11924=CARTESIAN_POINT('Ctrl Pts',(9.22738824529516,-0.528,-8.22742371893551));
#11925=CARTESIAN_POINT('',(9.22738824529516,0.,-8.22742371893551));
#11926=CARTESIAN_POINT('Ctrl Pts',(21.0225256793385,0.,-7.04790997553116));
#11927=CARTESIAN_POINT('Ctrl Pts',(19.8072013377325,0.,-4.22629716477465));
#11928=CARTESIAN_POINT('Ctrl Pts',(14.6387365156322,0.,-3.68706222835893));
#11929=CARTESIAN_POINT('Ctrl Pts',(9.29823038687031,0.,-5.29769106666559));
#11930=CARTESIAN_POINT('Ctrl Pts',(9.22738824529516,0.,-8.22742371893551));
#11931=CARTESIAN_POINT('',(9.22738824529516,1.2,-8.22742371893551));
#11932=CARTESIAN_POINT('',(9.22738824529516,1.2,-8.22742371893551));
#11933=CARTESIAN_POINT('Ctrl Pts',(21.0225256793385,1.2,-7.04790997553116));
#11934=CARTESIAN_POINT('Ctrl Pts',(19.8072013377325,1.2,-4.22629716477465));
#11935=CARTESIAN_POINT('Ctrl Pts',(14.6387365156322,1.2,-3.68706222835893));
#11936=CARTESIAN_POINT('Ctrl Pts',(9.29823038687031,1.2,-5.29769106666559));
#11937=CARTESIAN_POINT('Ctrl Pts',(9.22738824529516,1.2,-8.22742371893551));
#11938=CARTESIAN_POINT('Ctrl Pts',(9.22738824529516,1.2,-8.22742371893551));
#11939=CARTESIAN_POINT('Ctrl Pts',(9.22738824529516,-0.528,-8.22742371893551));
#11940=CARTESIAN_POINT('Ctrl Pts',(2.56764530386917,1.2,-8.25470956501187));
#11941=CARTESIAN_POINT('Ctrl Pts',(2.56764530386917,-0.528,-8.25470956501187));
#11942=CARTESIAN_POINT('Ctrl Pts',(-6.44753895416279,1.2,-9.5997804768992));
#11943=CARTESIAN_POINT('Ctrl Pts',(-6.44753895416279,-0.528,-9.5997804768992));
#11944=CARTESIAN_POINT('Ctrl Pts',(-18.1106375247657,1.2,-9.04522729065686));
#11945=CARTESIAN_POINT('Ctrl Pts',(-18.1106375247657,-0.528,-9.04522729065686));
#11946=CARTESIAN_POINT('Ctrl Pts',(-24.3161185416941,1.2,-8.46111575838443));
#11947=CARTESIAN_POINT('Ctrl Pts',(-24.3161185416941,-0.528,-8.46111575838443));
#11948=CARTESIAN_POINT('Ctrl Pts',(-28.8091126301565,1.2,-2.58884095234907));
#11949=CARTESIAN_POINT('Ctrl Pts',(-28.8091126301565,-0.528,-2.58884095234907));
#11950=CARTESIAN_POINT('Ctrl Pts',(-28.2500418808543,1.2,-2.07888836971769));
#11951=CARTESIAN_POINT('Ctrl Pts',(-28.2500418808543,-0.528,-2.07888836971769));
#11952=CARTESIAN_POINT('Ctrl Pts',(9.22738824529516,0.,-8.22742371893551));
#11953=CARTESIAN_POINT('Ctrl Pts',(2.56764530386917,0.,-8.25470956501187));
#11954=CARTESIAN_POINT('Ctrl Pts',(-6.44753895416279,0.,-9.5997804768992));
#11955=CARTESIAN_POINT('Ctrl Pts',(-18.1106375247657,0.,-9.04522729065686));
#11956=CARTESIAN_POINT('Ctrl Pts',(-24.3161185416941,0.,-8.46111575838443));
#11957=CARTESIAN_POINT('Ctrl Pts',(-28.8091126301565,0.,-2.58884095234907));
#11958=CARTESIAN_POINT('Ctrl Pts',(-28.2500418808543,0.,-2.07888836971769));
#11959=CARTESIAN_POINT('Ctrl Pts',(9.22738824529516,1.2,-8.22742371893551));
#11960=CARTESIAN_POINT('Ctrl Pts',(2.56764530386917,1.2,-8.25470956501187));
#11961=CARTESIAN_POINT('Ctrl Pts',(-6.44753895416279,1.2,-9.5997804768992));
#11962=CARTESIAN_POINT('Ctrl Pts',(-18.1106375247657,1.2,-9.04522729065686));
#11963=CARTESIAN_POINT('Ctrl Pts',(-24.3161185416941,1.2,-8.46111575838443));
#11964=CARTESIAN_POINT('Ctrl Pts',(-28.8091126301565,1.2,-2.58884095234907));
#11965=CARTESIAN_POINT('Ctrl Pts',(-28.2500418808543,1.2,-2.07888836971769));
#11966=CARTESIAN_POINT('Origin',(-2.41972159644388,1.2,5.11593538763785));
#11967=CARTESIAN_POINT('Origin',(-2.41972159644388,0.,5.11593538763785));
#12119=UNCERTAINTY_MEASURE_WITH_UNIT(LENGTH_MEASURE(0.01),#12138,
'DISTANCE_ACCURACY_VALUE',
'Maximum model space distance between geometric entities at asserted c
onnectivities');
#12123=UNCERTAINTY_MEASURE_WITH_UNIT(LENGTH_MEASURE(0.01),#12138,
'DISTANCE_ACCURACY_VALUE',
'Maximum model space distance between geometric entities at asserted c
onnectivities');
#12133=(
GEOMETRIC_REPRESENTATION_CONTEXT(3)
GLOBAL_UNCERTAINTY_ASSIGNED_CONTEXT((#12119))
GLOBAL_UNIT_ASSIGNED_CONTEXT((#12138,#12140,#12141))
REPRESENTATION_CONTEXT('','3D')
);
#12137=(
GEOMETRIC_REPRESENTATION_CONTEXT(3)
GLOBAL_UNCERTAINTY_ASSIGNED_CONTEXT((#12123))
GLOBAL_UNIT_ASSIGNED_CONTEXT((#12138,#12140,#12141))
REPRESENTATION_CONTEXT('','3D')
);
#12138=(
LENGTH_UNIT()
NAMED_UNIT(*)
SI_UNIT(.MILLI.,.METRE.)
);
#12140=(
NAMED_UNIT(*)
PLANE_ANGLE_UNIT()
SI_UNIT($,.RADIAN.)
);
#12141=(
NAMED_UNIT(*)
SI_UNIT($,.STERADIAN.)
SOLID_ANGLE_UNIT()
);
#12151=SHAPE_DEFINITION_REPRESENTATION(#12167,#12192);
#12167=PRODUCT_DEFINITION_SHAPE('',$,#12206);
#12192=SHAPE_REPRESENTATION('',(#2074),#12133);
#12196=PRODUCT_DEFINITION_CONTEXT('part definition',#12237,'design');
#12206=PRODUCT_DEFINITION('Bottol opener','Bottle opener',#12219,#12196);
#12219=PRODUCT_DEFINITION_FORMATION('',$,#12248);
#12237=APPLICATION_CONTEXT(
'Core Data for Automotive Mechanical Design Process');
#12238=PRODUCT_CONTEXT('part definition',#12237,'mechanical');
#12248=PRODUCT('Bottol opener','Bottle opener',$,(#12238));
#12253=PRESENTATION_STYLE_ASSIGNMENT((#12255));
#12255=SURFACE_STYLE_USAGE(.BOTH.,#12257);
#12257=SURFACE_SIDE_STYLE('',(#12259));
#12259=SURFACE_STYLE_FILL_AREA(#12261);
#12261=FILL_AREA_STYLE('Opaque(23,69,131)',(#12263));
#12263=FILL_AREA_STYLE_COLOUR('Opaque(23,69,131)',#12265);
#12265=COLOUR_RGB('Opaque(23,69,131)',0.0901960784313725,0.270588235294118,
0.513725490196078);
ENDSEC;
END-ISO-10303-21;
